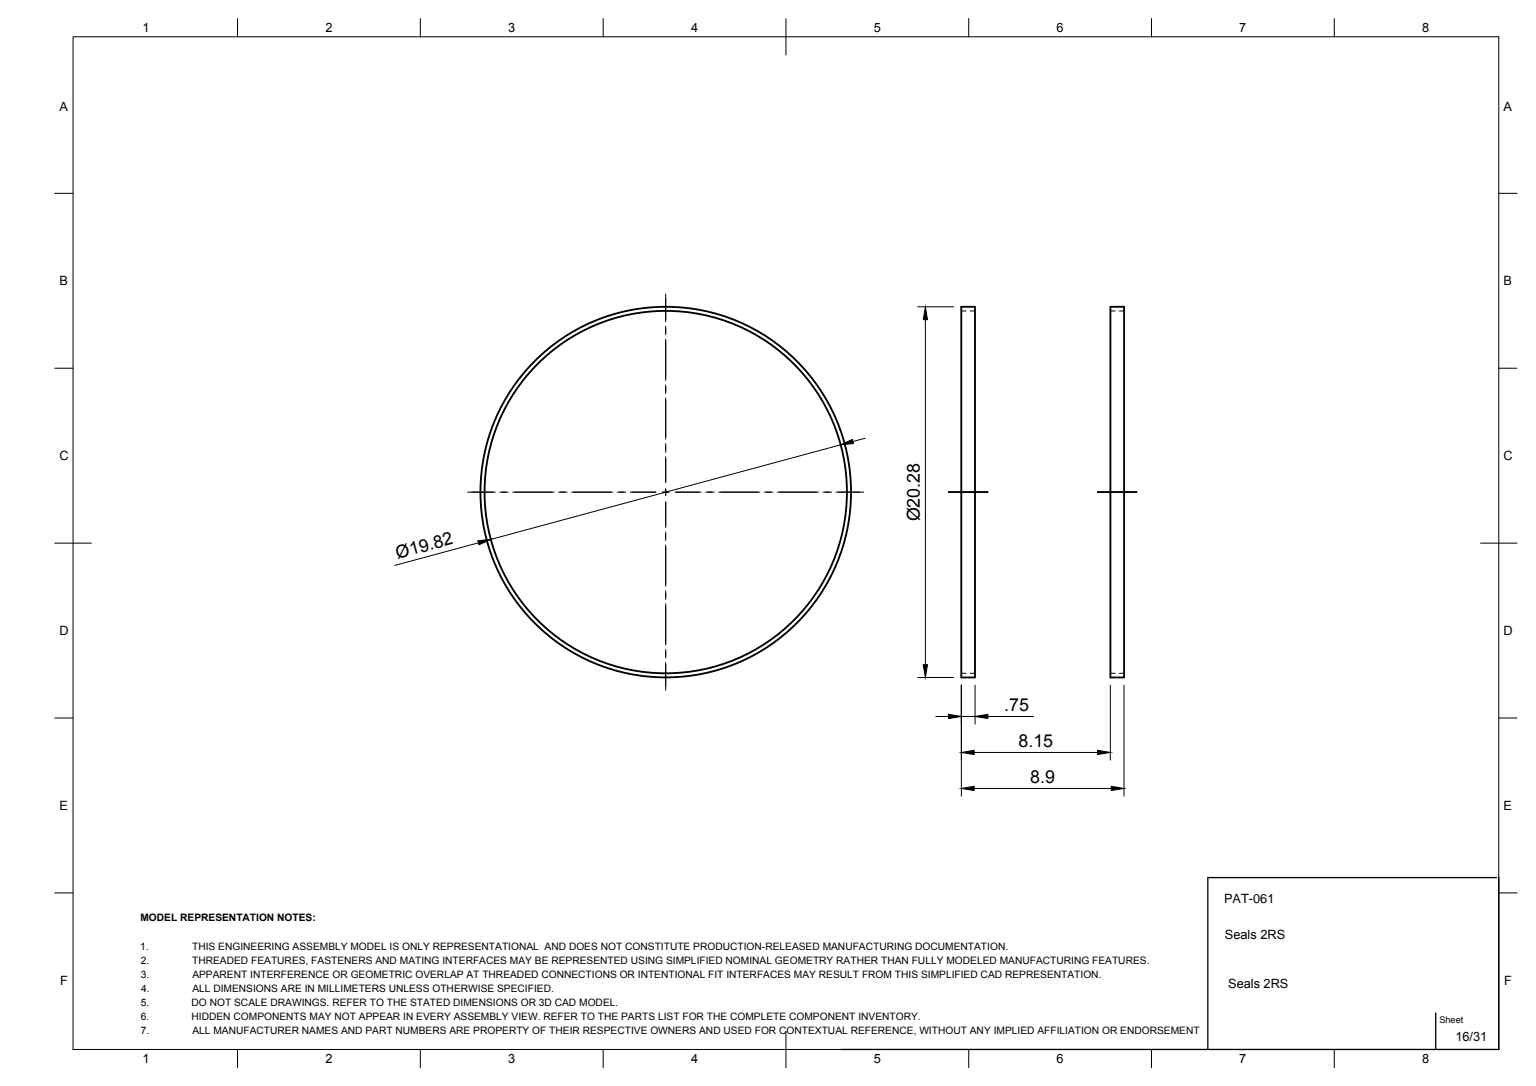
ISO-10303-21;
HEADER;
/* Generated by software containing ST-Developer
 * from STEP Tools, Inc. (www.steptools.com) 
 */

FILE_DESCRIPTION(
/* description */ ('Compact intermittent indexer'),
/* implementation_level */ '2;1');

FILE_NAME(
/* name */ 'Seals 2RS.step',
/* time_stamp */ '2026-10-29T16:32:17-07:00',
/* author */ (''),
/* organization */ (''),
/* preprocessor_version */ 'ST-DEVELOPER v20.2',
/* originating_system */ 'Autodesk Translation Framework v15.17.0.0',
/* authorisation */ '');

FILE_SCHEMA (('AUTOMOTIVE_DESIGN { 1 0 10303 214 3 1 1 }'));
ENDSEC;

DATA;
#10=MECHANICAL_DESIGN_GEOMETRIC_PRESENTATION_REPRESENTATION('',(#274,#275),#10837);
#219=SHAPE_REPRESENTATION_RELATIONSHIP('SRR','None',#10954,#243);
#243=ADVANCED_BREP_SHAPE_REPRESENTATION('',(#305,#306),#10821);
#274=STYLED_ITEM('',(#11166),#305);
#275=STYLED_ITEM('',(#11166),#306);
#305=MANIFOLD_SOLID_BREP('Body1',#5647);
#306=MANIFOLD_SOLID_BREP('Body2',#5648);
#428=FACE_BOUND('',#1225,.T.);
#429=FACE_BOUND('',#1228,.T.);
#430=FACE_BOUND('',#1231,.T.);
#431=FACE_BOUND('',#1234,.T.);
#552=PLANE('',#6301);
#553=PLANE('',#6306);
#554=PLANE('',#6309);
#555=PLANE('',#6314);
#821=FACE_OUTER_BOUND('',#1224,.T.);
#822=FACE_OUTER_BOUND('',#1226,.T.);
#823=FACE_OUTER_BOUND('',#1227,.T.);
#824=FACE_OUTER_BOUND('',#1229,.T.);
#825=FACE_OUTER_BOUND('',#1230,.T.);
#826=FACE_OUTER_BOUND('',#1232,.T.);
#827=FACE_OUTER_BOUND('',#1233,.T.);
#828=FACE_OUTER_BOUND('',#1235,.T.);
#1224=EDGE_LOOP('',(#4416));
#1225=EDGE_LOOP('',(#4417));
#1226=EDGE_LOOP('',(#4418,#4419,#4420,#4421));
#1227=EDGE_LOOP('',(#4422));
#1228=EDGE_LOOP('',(#4423));
#1229=EDGE_LOOP('',(#4424,#4425,#4426,#4427));
#1230=EDGE_LOOP('',(#4428));
#1231=EDGE_LOOP('',(#4429));
#1232=EDGE_LOOP('',(#4430,#4431,#4432,#4433));
#1233=EDGE_LOOP('',(#4434));
#1234=EDGE_LOOP('',(#4435));
#1235=EDGE_LOOP('',(#4436,#4437,#4438,#4439));
#1576=LINE('',#9693,#1934);
#1577=LINE('',#9698,#1935);
#1578=LINE('',#9707,#1936);
#1579=LINE('',#9712,#1937);
#1934=VECTOR('',#7566,1.013815);
#1935=VECTOR('',#7573,0.991185);
#1936=VECTOR('',#7584,1.013815);
#1937=VECTOR('',#7591,0.991185);
#2338=CIRCLE('',#6302,1.013815);
#2339=CIRCLE('',#6303,0.991185);
#2340=CIRCLE('',#6305,1.013815);
#2341=CIRCLE('',#6307,0.991185);
#2342=CIRCLE('',#6310,1.013815);
#2343=CIRCLE('',#6311,0.991185);
#2344=CIRCLE('',#6313,1.013815);
#2345=CIRCLE('',#6315,0.991185);
#2726=VERTEX_POINT('',#9686);
#2727=VERTEX_POINT('',#9688);
#2728=VERTEX_POINT('',#9691);
#2729=VERTEX_POINT('',#9695);
#2730=VERTEX_POINT('',#9700);
#2731=VERTEX_POINT('',#9702);
#2732=VERTEX_POINT('',#9705);
#2733=VERTEX_POINT('',#9709);
#3330=EDGE_CURVE('',#2726,#2726,#2338,.T.);
#3331=EDGE_CURVE('',#2727,#2727,#2339,.T.);
#3332=EDGE_CURVE('',#2728,#2728,#2340,.T.);
#3333=EDGE_CURVE('',#2728,#2726,#1576,.T.);
#3334=EDGE_CURVE('',#2729,#2729,#2341,.T.);
#3335=EDGE_CURVE('',#2729,#2727,#1577,.T.);
#3336=EDGE_CURVE('',#2730,#2730,#2342,.T.);
#3337=EDGE_CURVE('',#2731,#2731,#2343,.T.);
#3338=EDGE_CURVE('',#2732,#2732,#2344,.T.);
#3339=EDGE_CURVE('',#2732,#2730,#1578,.T.);
#3340=EDGE_CURVE('',#2733,#2733,#2345,.T.);
#3341=EDGE_CURVE('',#2733,#2731,#1579,.T.);
#4416=ORIENTED_EDGE('',*,*,#3330,.F.);
#4417=ORIENTED_EDGE('',*,*,#3331,.T.);
#4418=ORIENTED_EDGE('',*,*,#3332,.F.);
#4419=ORIENTED_EDGE('',*,*,#3333,.T.);
#4420=ORIENTED_EDGE('',*,*,#3330,.T.);
#4421=ORIENTED_EDGE('',*,*,#3333,.F.);
#4422=ORIENTED_EDGE('',*,*,#3332,.T.);
#4423=ORIENTED_EDGE('',*,*,#3334,.F.);
#4424=ORIENTED_EDGE('',*,*,#3334,.T.);
#4425=ORIENTED_EDGE('',*,*,#3335,.T.);
#4426=ORIENTED_EDGE('',*,*,#3331,.F.);
#4427=ORIENTED_EDGE('',*,*,#3335,.F.);
#4428=ORIENTED_EDGE('',*,*,#3336,.F.);
#4429=ORIENTED_EDGE('',*,*,#3337,.T.);
#4430=ORIENTED_EDGE('',*,*,#3338,.F.);
#4431=ORIENTED_EDGE('',*,*,#3339,.T.);
#4432=ORIENTED_EDGE('',*,*,#3336,.T.);
#4433=ORIENTED_EDGE('',*,*,#3339,.F.);
#4434=ORIENTED_EDGE('',*,*,#3338,.T.);
#4435=ORIENTED_EDGE('',*,*,#3340,.F.);
#4436=ORIENTED_EDGE('',*,*,#3340,.T.);
#4437=ORIENTED_EDGE('',*,*,#3341,.T.);
#4438=ORIENTED_EDGE('',*,*,#3337,.F.);
#4439=ORIENTED_EDGE('',*,*,#3341,.F.);
#5234=CYLINDRICAL_SURFACE('',#6304,1.013815);
#5235=CYLINDRICAL_SURFACE('',#6308,0.991185);
#5236=CYLINDRICAL_SURFACE('',#6312,1.013815);
#5237=CYLINDRICAL_SURFACE('',#6316,0.991185);
#5464=ADVANCED_FACE('',(#821,#428),#552,.T.);
#5465=ADVANCED_FACE('',(#822),#5234,.T.);
#5466=ADVANCED_FACE('',(#823,#429),#553,.T.);
#5467=ADVANCED_FACE('',(#824),#5235,.F.);
#5468=ADVANCED_FACE('',(#825,#430),#554,.T.);
#5469=ADVANCED_FACE('',(#826),#5236,.T.);
#5470=ADVANCED_FACE('',(#827,#431),#555,.T.);
#5471=ADVANCED_FACE('',(#828),#5237,.F.);
#5647=CLOSED_SHELL('',(#5464,#5465,#5466,#5467));
#5648=CLOSED_SHELL('',(#5468,#5469,#5470,#5471));
#6300=AXIS2_PLACEMENT_3D('',#9684,#7554,#7555);
#6301=AXIS2_PLACEMENT_3D('',#9685,#7556,#7557);
#6302=AXIS2_PLACEMENT_3D('',#9687,#7558,#7559);
#6303=AXIS2_PLACEMENT_3D('',#9689,#7560,#7561);
#6304=AXIS2_PLACEMENT_3D('',#9690,#7562,#7563);
#6305=AXIS2_PLACEMENT_3D('',#9692,#7564,#7565);
#6306=AXIS2_PLACEMENT_3D('',#9694,#7567,#7568);
#6307=AXIS2_PLACEMENT_3D('',#9696,#7569,#7570);
#6308=AXIS2_PLACEMENT_3D('',#9697,#7571,#7572);
#6309=AXIS2_PLACEMENT_3D('',#9699,#7574,#7575);
#6310=AXIS2_PLACEMENT_3D('',#9701,#7576,#7577);
#6311=AXIS2_PLACEMENT_3D('',#9703,#7578,#7579);
#6312=AXIS2_PLACEMENT_3D('',#9704,#7580,#7581);
#6313=AXIS2_PLACEMENT_3D('',#9706,#7582,#7583);
#6314=AXIS2_PLACEMENT_3D('',#9708,#7585,#7586);
#6315=AXIS2_PLACEMENT_3D('',#9710,#7587,#7588);
#6316=AXIS2_PLACEMENT_3D('',#9711,#7589,#7590);
#7554=DIRECTION('axis',(0.,0.,1.));
#7555=DIRECTION('refdir',(1.,0.,0.));
#7556=DIRECTION('center_axis',(0.,1.,0.));
#7557=DIRECTION('ref_axis',(0.,0.,1.));
#7558=DIRECTION('center_axis',(0.,-1.,0.));
#7559=DIRECTION('ref_axis',(1.,0.,0.));
#7560=DIRECTION('center_axis',(0.,-1.,0.));
#7561=DIRECTION('ref_axis',(1.,0.,0.));
#7562=DIRECTION('center_axis',(0.,-1.,0.));
#7563=DIRECTION('ref_axis',(1.,0.,0.));
#7564=DIRECTION('center_axis',(0.,-1.,0.));
#7565=DIRECTION('ref_axis',(1.,0.,0.));
#7566=DIRECTION('',(0.,1.,0.));
#7567=DIRECTION('center_axis',(0.,-1.,0.));
#7568=DIRECTION('ref_axis',(0.,0.,-1.));
#7569=DIRECTION('center_axis',(0.,-1.,0.));
#7570=DIRECTION('ref_axis',(1.,0.,0.));
#7571=DIRECTION('center_axis',(0.,-1.,0.));
#7572=DIRECTION('ref_axis',(1.,0.,0.));
#7573=DIRECTION('',(0.,1.,0.));
#7574=DIRECTION('center_axis',(0.,1.,0.));
#7575=DIRECTION('ref_axis',(0.,0.,1.));
#7576=DIRECTION('center_axis',(0.,-1.,0.));
#7577=DIRECTION('ref_axis',(1.,0.,0.));
#7578=DIRECTION('center_axis',(0.,-1.,0.));
#7579=DIRECTION('ref_axis',(1.,0.,0.));
#7580=DIRECTION('center_axis',(0.,-1.,0.));
#7581=DIRECTION('ref_axis',(1.,0.,0.));
#7582=DIRECTION('center_axis',(0.,-1.,0.));
#7583=DIRECTION('ref_axis',(1.,0.,0.));
#7584=DIRECTION('',(0.,1.,0.));
#7585=DIRECTION('center_axis',(0.,-1.,0.));
#7586=DIRECTION('ref_axis',(0.,0.,-1.));
#7587=DIRECTION('center_axis',(0.,-1.,0.));
#7588=DIRECTION('ref_axis',(1.,0.,0.));
#7589=DIRECTION('center_axis',(0.,-1.,0.));
#7590=DIRECTION('ref_axis',(1.,0.,0.));
#7591=DIRECTION('',(0.,1.,0.));
#9684=CARTESIAN_POINT('',(0.,0.,0.));
#9685=CARTESIAN_POINT('Origin',(1.013815,0.445,0.));
#9686=CARTESIAN_POINT('',(-1.013815,0.445,-1.24156529467757E-16));
#9687=CARTESIAN_POINT('Origin',(0.,0.445,0.));
#9688=CARTESIAN_POINT('',(-0.991185,0.445,-1.21385153761287E-16));
#9689=CARTESIAN_POINT('Origin',(0.,0.445,0.));
#9690=CARTESIAN_POINT('Origin',(0.,0.4075,0.));
#9691=CARTESIAN_POINT('',(-1.013815,0.37,-1.24156529467757E-16));
#9692=CARTESIAN_POINT('Origin',(0.,0.37,0.));
#9693=CARTESIAN_POINT('',(-1.013815,0.4075,-1.24156529467757E-16));
#9694=CARTESIAN_POINT('Origin',(0.991185,0.37,0.));
#9695=CARTESIAN_POINT('',(-0.991185,0.37,-1.21385153761287E-16));
#9696=CARTESIAN_POINT('Origin',(0.,0.37,0.));
#9697=CARTESIAN_POINT('Origin',(0.,0.4075,0.));
#9698=CARTESIAN_POINT('',(-0.991185,0.4075,-1.21385153761287E-16));
#9699=CARTESIAN_POINT('Origin',(1.013815,-0.37,0.));
#9700=CARTESIAN_POINT('',(-1.013815,-0.37,-1.24156529467757E-16));
#9701=CARTESIAN_POINT('Origin',(0.,-0.37,0.));
#9702=CARTESIAN_POINT('',(-0.991185,-0.37,-1.21385153761287E-16));
#9703=CARTESIAN_POINT('Origin',(0.,-0.37,0.));
#9704=CARTESIAN_POINT('Origin',(0.,-0.4075,0.));
#9705=CARTESIAN_POINT('',(-1.013815,-0.445,-1.24156529467757E-16));
#9706=CARTESIAN_POINT('Origin',(0.,-0.445,0.));
#9707=CARTESIAN_POINT('',(-1.013815,-0.4075,-1.24156529467757E-16));
#9708=CARTESIAN_POINT('Origin',(0.991185,-0.445,0.));
#9709=CARTESIAN_POINT('',(-0.991185,-0.445,-1.21385153761287E-16));
#9710=CARTESIAN_POINT('Origin',(0.,-0.445,0.));
#9711=CARTESIAN_POINT('Origin',(0.,-0.4075,0.));
#9712=CARTESIAN_POINT('',(-0.991185,-0.4075,-1.21385153761287E-16));
#10791=UNCERTAINTY_MEASURE_WITH_UNIT(LENGTH_MEASURE(0.001),#10838,
'DISTANCE_ACCURACY_VALUE',
'Maximum model space distance between geometric entities at asserted c
onnectivities');
#10807=UNCERTAINTY_MEASURE_WITH_UNIT(LENGTH_MEASURE(0.001),#10838,
'DISTANCE_ACCURACY_VALUE',
'Maximum model space distance between geometric entities at asserted c
onnectivities');
#10821=(
GEOMETRIC_REPRESENTATION_CONTEXT(3)
GLOBAL_UNCERTAINTY_ASSIGNED_CONTEXT((#10791))
GLOBAL_UNIT_ASSIGNED_CONTEXT((#10838,#10840,#10841))
REPRESENTATION_CONTEXT('','3D')
);
#10837=(
GEOMETRIC_REPRESENTATION_CONTEXT(3)
GLOBAL_UNCERTAINTY_ASSIGNED_CONTEXT((#10807))
GLOBAL_UNIT_ASSIGNED_CONTEXT((#10838,#10840,#10841))
REPRESENTATION_CONTEXT('','3D')
);
#10838=(
LENGTH_UNIT()
NAMED_UNIT(*)
SI_UNIT(.CENTI.,.METRE.)
);
#10840=(
NAMED_UNIT(*)
PLANE_ANGLE_UNIT()
SI_UNIT($,.RADIAN.)
);
#10841=(
NAMED_UNIT(*)
SI_UNIT($,.STERADIAN.)
SOLID_ANGLE_UNIT()
);
#10855=SHAPE_DEFINITION_REPRESENTATION(#10884,#10954);
#10884=PRODUCT_DEFINITION_SHAPE('',$,#10984);
#10954=SHAPE_REPRESENTATION('',(#6300),#10821);
#10970=PRODUCT_DEFINITION_CONTEXT('part definition',#11059,'design');
#10984=PRODUCT_DEFINITION('Seals 2RS','Seals 2RS',#11013,#10970);
#11013=PRODUCT_DEFINITION_FORMATION('',$,#11074);
#11059=APPLICATION_CONTEXT(
'Core Data for Automotive Mechanical Design Process');
#11060=PRODUCT_CONTEXT('part definition',#11059,'mechanical');
#11074=PRODUCT('Seals 2RS','Seals 2RS','Seals 2RS',(#11060));
#11160=COLOUR_RGB('Grey',0.48,0.52,0.57);
#11161=FILL_AREA_STYLE_COLOUR('',#11160);
#11162=FILL_AREA_STYLE('',(#11161));
#11163=SURFACE_STYLE_FILL_AREA(#11162);
#11164=SURFACE_SIDE_STYLE('',(#11163));
#11165=SURFACE_STYLE_USAGE(.BOTH.,#11164);
#11166=PRESENTATION_STYLE_ASSIGNMENT((#11165));
ENDSEC;
END-ISO-10303-21;
